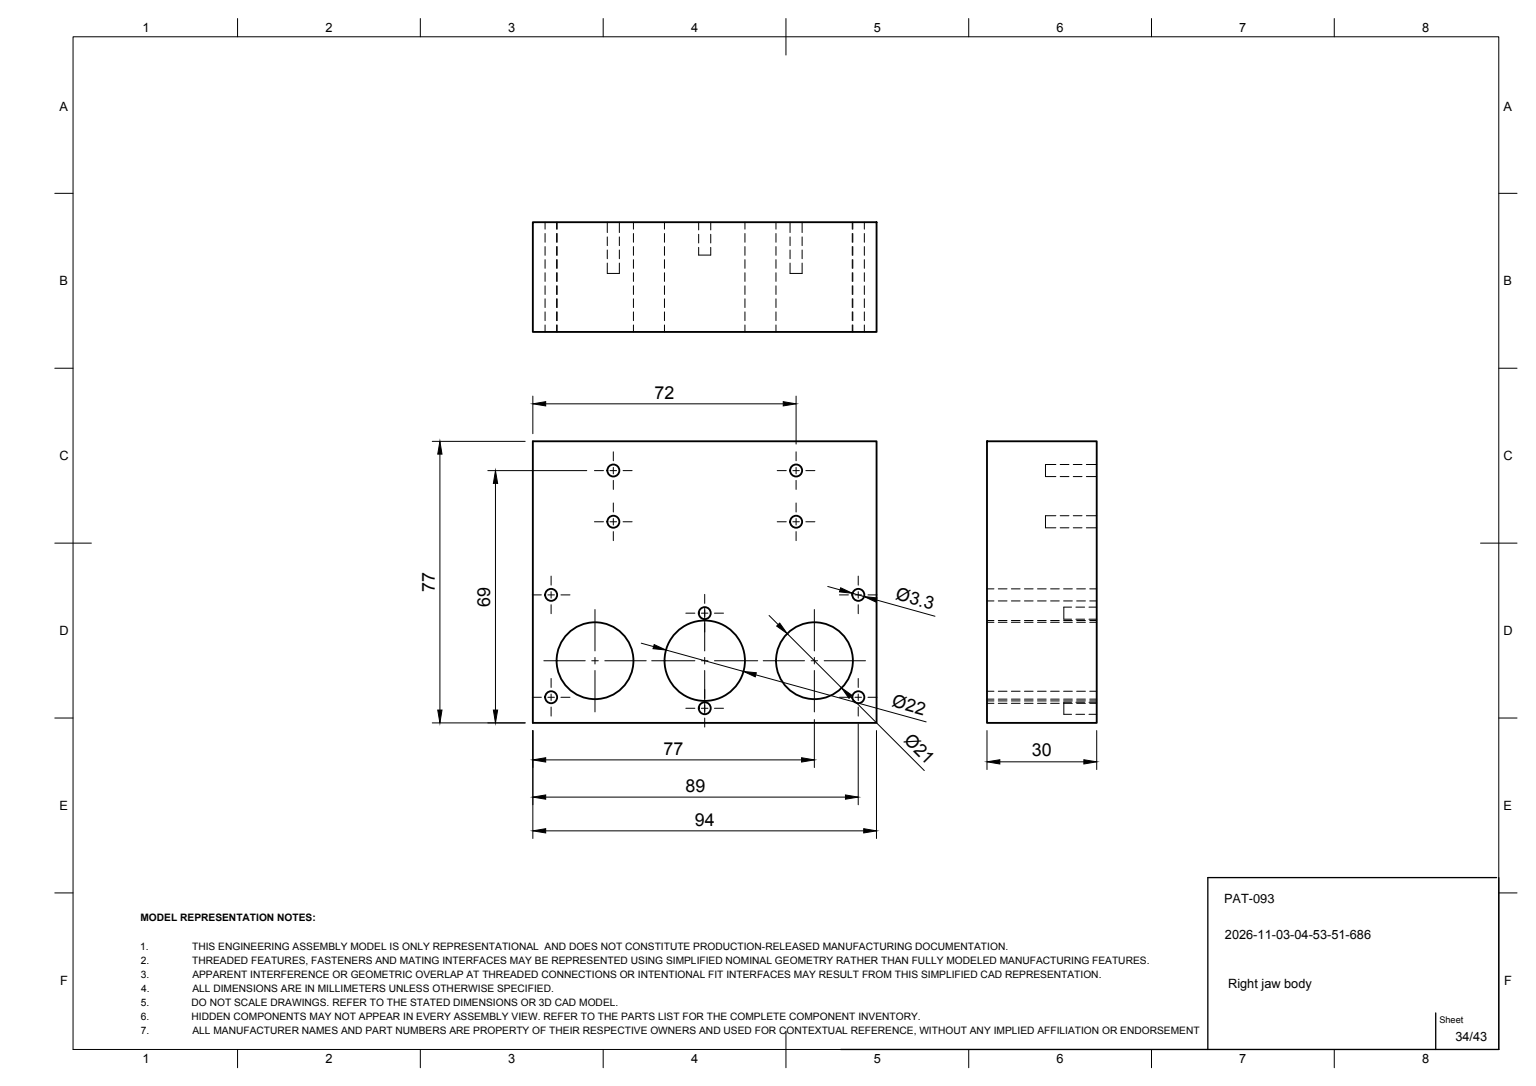
ISO-10303-21;
HEADER;
/* Generated by software containing ST-Developer
 * from STEP Tools, Inc. (www.steptools.com) 
 */

FILE_DESCRIPTION(
/* description */ ('Self-centering screw clamp'),
/* implementation_level */ '2;1');

FILE_NAME(
/* name */ 'Right jaw body.step',
/* time_stamp */ '2026-10-28T03:25:31-07:00',
/* author */ (''),
/* organization */ (''),
/* preprocessor_version */ 'ST-DEVELOPER v20.2',
/* originating_system */ 'Autodesk Translation Framework v15.17.0.0',
/* authorisation */ '');

FILE_SCHEMA (('AUTOMOTIVE_DESIGN { 1 0 10303 214 3 1 1 }'));
ENDSEC;

DATA;
#10=MECHANICAL_DESIGN_GEOMETRIC_PRESENTATION_REPRESENTATION('',(#655),#16799);
#566=SHAPE_REPRESENTATION_RELATIONSHIP('SRR','None',#17042,#607);
#607=ADVANCED_BREP_SHAPE_REPRESENTATION('',(#703),#16780);
#655=STYLED_ITEM('',(#17305),#703);
#703=MANIFOLD_SOLID_BREP('Body1',#9106);
#916=FACE_BOUND('',#2304,.T.);
#917=FACE_BOUND('',#2305,.T.);
#918=FACE_BOUND('',#2306,.T.);
#919=FACE_BOUND('',#2307,.T.);
#920=FACE_BOUND('',#2308,.T.);
#921=FACE_BOUND('',#2309,.T.);
#922=FACE_BOUND('',#2310,.T.);
#923=FACE_BOUND('',#2313,.T.);
#924=FACE_BOUND('',#2314,.T.);
#925=FACE_BOUND('',#2315,.T.);
#926=FACE_BOUND('',#2316,.T.);
#927=FACE_BOUND('',#2317,.T.);
#928=FACE_BOUND('',#2318,.T.);
#929=FACE_BOUND('',#2319,.T.);
#930=FACE_BOUND('',#2320,.T.);
#931=FACE_BOUND('',#2321,.T.);
#932=FACE_BOUND('',#2322,.T.);
#933=FACE_BOUND('',#2323,.T.);
#934=FACE_BOUND('',#2324,.T.);
#935=FACE_BOUND('',#2325,.T.);
#1161=PLANE('',#10260);
#1162=PLANE('',#10264);
#1163=PLANE('',#10268);
#1164=PLANE('',#10272);
#1165=PLANE('',#10276);
#1166=PLANE('',#10280);
#1167=PLANE('',#10302);
#1168=PLANE('',#10303);
#1169=PLANE('',#10304);
#1170=PLANE('',#10305);
#1171=PLANE('',#10306);
#1172=PLANE('',#10307);
#1581=FACE_OUTER_BOUND('',#2283,.T.);
#1582=FACE_OUTER_BOUND('',#2284,.T.);
#1583=FACE_OUTER_BOUND('',#2285,.T.);
#1584=FACE_OUTER_BOUND('',#2286,.T.);
#1585=FACE_OUTER_BOUND('',#2287,.T.);
#1586=FACE_OUTER_BOUND('',#2288,.T.);
#1587=FACE_OUTER_BOUND('',#2289,.T.);
#1588=FACE_OUTER_BOUND('',#2290,.T.);
#1589=FACE_OUTER_BOUND('',#2291,.T.);
#1590=FACE_OUTER_BOUND('',#2292,.T.);
#1591=FACE_OUTER_BOUND('',#2293,.T.);
#1592=FACE_OUTER_BOUND('',#2294,.T.);
#1593=FACE_OUTER_BOUND('',#2295,.T.);
#1594=FACE_OUTER_BOUND('',#2296,.T.);
#1595=FACE_OUTER_BOUND('',#2297,.T.);
#1596=FACE_OUTER_BOUND('',#2298,.T.);
#1597=FACE_OUTER_BOUND('',#2299,.T.);
#1598=FACE_OUTER_BOUND('',#2300,.T.);
#1599=FACE_OUTER_BOUND('',#2301,.T.);
#1600=FACE_OUTER_BOUND('',#2302,.T.);
#1601=FACE_OUTER_BOUND('',#2303,.T.);
#1602=FACE_OUTER_BOUND('',#2311,.T.);
#1603=FACE_OUTER_BOUND('',#2312,.T.);
#1604=FACE_OUTER_BOUND('',#2326,.T.);
#1605=FACE_OUTER_BOUND('',#2327,.T.);
#2283=EDGE_LOOP('',(#7551,#7552,#7553,#7554));
#2284=EDGE_LOOP('',(#7555));
#2285=EDGE_LOOP('',(#7556,#7557,#7558,#7559));
#2286=EDGE_LOOP('',(#7560));
#2287=EDGE_LOOP('',(#7561,#7562,#7563,#7564));
#2288=EDGE_LOOP('',(#7565));
#2289=EDGE_LOOP('',(#7566,#7567,#7568,#7569));
#2290=EDGE_LOOP('',(#7570));
#2291=EDGE_LOOP('',(#7571,#7572,#7573,#7574));
#2292=EDGE_LOOP('',(#7575));
#2293=EDGE_LOOP('',(#7576,#7577,#7578,#7579));
#2294=EDGE_LOOP('',(#7580));
#2295=EDGE_LOOP('',(#7581,#7582,#7583,#7584));
#2296=EDGE_LOOP('',(#7585,#7586,#7587,#7588));
#2297=EDGE_LOOP('',(#7589,#7590,#7591,#7592));
#2298=EDGE_LOOP('',(#7593,#7594,#7595,#7596));
#2299=EDGE_LOOP('',(#7597,#7598,#7599,#7600));
#2300=EDGE_LOOP('',(#7601,#7602,#7603,#7604));
#2301=EDGE_LOOP('',(#7605,#7606,#7607,#7608));
#2302=EDGE_LOOP('',(#7609,#7610,#7611,#7612));
#2303=EDGE_LOOP('',(#7613,#7614,#7615,#7616));
#2304=EDGE_LOOP('',(#7617));
#2305=EDGE_LOOP('',(#7618));
#2306=EDGE_LOOP('',(#7619));
#2307=EDGE_LOOP('',(#7620));
#2308=EDGE_LOOP('',(#7621));
#2309=EDGE_LOOP('',(#7622));
#2310=EDGE_LOOP('',(#7623));
#2311=EDGE_LOOP('',(#7624,#7625,#7626,#7627));
#2312=EDGE_LOOP('',(#7628,#7629,#7630,#7631));
#2313=EDGE_LOOP('',(#7632));
#2314=EDGE_LOOP('',(#7633));
#2315=EDGE_LOOP('',(#7634));
#2316=EDGE_LOOP('',(#7635));
#2317=EDGE_LOOP('',(#7636));
#2318=EDGE_LOOP('',(#7637));
#2319=EDGE_LOOP('',(#7638));
#2320=EDGE_LOOP('',(#7639));
#2321=EDGE_LOOP('',(#7640));
#2322=EDGE_LOOP('',(#7641));
#2323=EDGE_LOOP('',(#7642));
#2324=EDGE_LOOP('',(#7643));
#2325=EDGE_LOOP('',(#7644));
#2326=EDGE_LOOP('',(#7645,#7646,#7647,#7648));
#2327=EDGE_LOOP('',(#7649,#7650,#7651,#7652));
#2934=LINE('',#15598,#3507);
#2935=LINE('',#15605,#3508);
#2936=LINE('',#15612,#3509);
#2937=LINE('',#15619,#3510);
#2938=LINE('',#15626,#3511);
#2939=LINE('',#15633,#3512);
#2940=LINE('',#15640,#3513);
#2941=LINE('',#15646,#3514);
#2942=LINE('',#15652,#3515);
#2943=LINE('',#15658,#3516);
#2944=LINE('',#15664,#3517);
#2945=LINE('',#15670,#3518);
#2946=LINE('',#15676,#3519);
#2947=LINE('',#15681,#3520);
#2948=LINE('',#15683,#3521);
#2949=LINE('',#15685,#3522);
#2950=LINE('',#15686,#3523);
#2951=LINE('',#15689,#3524);
#2952=LINE('',#15691,#3525);
#2953=LINE('',#15692,#3526);
#2954=LINE('',#15695,#3527);
#2955=LINE('',#15697,#3528);
#2956=LINE('',#15698,#3529);
#2957=LINE('',#15700,#3530);
#2958=LINE('',#15701,#3531);
#3507=VECTOR('',#12473,0.165);
#3508=VECTOR('',#12482,0.164999999999999);
#3509=VECTOR('',#12491,0.165);
#3510=VECTOR('',#12500,0.164999999999999);
#3511=VECTOR('',#12509,0.165);
#3512=VECTOR('',#12518,0.165);
#3513=VECTOR('',#12527,0.165);
#3514=VECTOR('',#12534,0.165);
#3515=VECTOR('',#12541,0.165);
#3516=VECTOR('',#12548,0.165);
#3517=VECTOR('',#12555,1.1);
#3518=VECTOR('',#12562,1.05);
#3519=VECTOR('',#12569,1.05);
#3520=VECTOR('',#12574,1.);
#3521=VECTOR('',#12575,1.);
#3522=VECTOR('',#12576,1.);
#3523=VECTOR('',#12577,1.);
#3524=VECTOR('',#12580,1.);
#3525=VECTOR('',#12581,1.);
#3526=VECTOR('',#12582,1.);
#3527=VECTOR('',#12585,1.);
#3528=VECTOR('',#12586,1.);
#3529=VECTOR('',#12587,1.);
#3530=VECTOR('',#12590,1.);
#3531=VECTOR('',#12591,1.);
#4060=CIRCLE('',#10258,0.165);
#4061=CIRCLE('',#10259,0.165);
#4062=CIRCLE('',#10262,0.164999999999999);
#4063=CIRCLE('',#10263,0.164999999999999);
#4064=CIRCLE('',#10266,0.165);
#4065=CIRCLE('',#10267,0.165);
#4066=CIRCLE('',#10270,0.164999999999999);
#4067=CIRCLE('',#10271,0.164999999999999);
#4068=CIRCLE('',#10274,0.165);
#4069=CIRCLE('',#10275,0.165);
#4070=CIRCLE('',#10278,0.165);
#4071=CIRCLE('',#10279,0.165);
#4072=CIRCLE('',#10282,0.165);
#4073=CIRCLE('',#10283,0.165);
#4074=CIRCLE('',#10285,0.165);
#4075=CIRCLE('',#10286,0.165);
#4076=CIRCLE('',#10288,0.165);
#4077=CIRCLE('',#10289,0.165);
#4078=CIRCLE('',#10291,0.165);
#4079=CIRCLE('',#10292,0.165);
#4080=CIRCLE('',#10294,1.1);
#4081=CIRCLE('',#10295,1.1);
#4082=CIRCLE('',#10297,1.05);
#4083=CIRCLE('',#10298,1.05);
#4084=CIRCLE('',#10300,1.05);
#4085=CIRCLE('',#10301,1.05);
#4711=VERTEX_POINT('',#15595);
#4712=VERTEX_POINT('',#15597);
#4713=VERTEX_POINT('',#15602);
#4714=VERTEX_POINT('',#15604);
#4715=VERTEX_POINT('',#15609);
#4716=VERTEX_POINT('',#15611);
#4717=VERTEX_POINT('',#15616);
#4718=VERTEX_POINT('',#15618);
#4719=VERTEX_POINT('',#15623);
#4720=VERTEX_POINT('',#15625);
#4721=VERTEX_POINT('',#15630);
#4722=VERTEX_POINT('',#15632);
#4723=VERTEX_POINT('',#15637);
#4724=VERTEX_POINT('',#15639);
#4725=VERTEX_POINT('',#15643);
#4726=VERTEX_POINT('',#15645);
#4727=VERTEX_POINT('',#15649);
#4728=VERTEX_POINT('',#15651);
#4729=VERTEX_POINT('',#15655);
#4730=VERTEX_POINT('',#15657);
#4731=VERTEX_POINT('',#15661);
#4732=VERTEX_POINT('',#15663);
#4733=VERTEX_POINT('',#15667);
#4734=VERTEX_POINT('',#15669);
#4735=VERTEX_POINT('',#15673);
#4736=VERTEX_POINT('',#15675);
#4737=VERTEX_POINT('',#15679);
#4738=VERTEX_POINT('',#15680);
#4739=VERTEX_POINT('',#15682);
#4740=VERTEX_POINT('',#15684);
#4741=VERTEX_POINT('',#15688);
#4742=VERTEX_POINT('',#15690);
#4743=VERTEX_POINT('',#15694);
#4744=VERTEX_POINT('',#15696);
#5700=EDGE_CURVE('',#4711,#4711,#4060,.T.);
#5701=EDGE_CURVE('',#4711,#4712,#2934,.T.);
#5702=EDGE_CURVE('',#4712,#4712,#4061,.T.);
#5703=EDGE_CURVE('',#4713,#4713,#4062,.T.);
#5704=EDGE_CURVE('',#4713,#4714,#2935,.T.);
#5705=EDGE_CURVE('',#4714,#4714,#4063,.T.);
#5706=EDGE_CURVE('',#4715,#4715,#4064,.T.);
#5707=EDGE_CURVE('',#4715,#4716,#2936,.T.);
#5708=EDGE_CURVE('',#4716,#4716,#4065,.T.);
#5709=EDGE_CURVE('',#4717,#4717,#4066,.T.);
#5710=EDGE_CURVE('',#4717,#4718,#2937,.T.);
#5711=EDGE_CURVE('',#4718,#4718,#4067,.T.);
#5712=EDGE_CURVE('',#4719,#4719,#4068,.T.);
#5713=EDGE_CURVE('',#4719,#4720,#2938,.T.);
#5714=EDGE_CURVE('',#4720,#4720,#4069,.T.);
#5715=EDGE_CURVE('',#4721,#4721,#4070,.T.);
#5716=EDGE_CURVE('',#4721,#4722,#2939,.T.);
#5717=EDGE_CURVE('',#4722,#4722,#4071,.T.);
#5718=EDGE_CURVE('',#4723,#4723,#4072,.T.);
#5719=EDGE_CURVE('',#4723,#4724,#2940,.T.);
#5720=EDGE_CURVE('',#4724,#4724,#4073,.T.);
#5721=EDGE_CURVE('',#4725,#4725,#4074,.T.);
#5722=EDGE_CURVE('',#4725,#4726,#2941,.T.);
#5723=EDGE_CURVE('',#4726,#4726,#4075,.T.);
#5724=EDGE_CURVE('',#4727,#4727,#4076,.T.);
#5725=EDGE_CURVE('',#4727,#4728,#2942,.T.);
#5726=EDGE_CURVE('',#4728,#4728,#4077,.T.);
#5727=EDGE_CURVE('',#4729,#4729,#4078,.T.);
#5728=EDGE_CURVE('',#4729,#4730,#2943,.T.);
#5729=EDGE_CURVE('',#4730,#4730,#4079,.T.);
#5730=EDGE_CURVE('',#4731,#4731,#4080,.T.);
#5731=EDGE_CURVE('',#4731,#4732,#2944,.T.);
#5732=EDGE_CURVE('',#4732,#4732,#4081,.T.);
#5733=EDGE_CURVE('',#4733,#4733,#4082,.T.);
#5734=EDGE_CURVE('',#4733,#4734,#2945,.T.);
#5735=EDGE_CURVE('',#4734,#4734,#4083,.T.);
#5736=EDGE_CURVE('',#4735,#4735,#4084,.T.);
#5737=EDGE_CURVE('',#4735,#4736,#2946,.T.);
#5738=EDGE_CURVE('',#4736,#4736,#4085,.T.);
#5739=EDGE_CURVE('',#4737,#4738,#2947,.T.);
#5740=EDGE_CURVE('',#4738,#4739,#2948,.T.);
#5741=EDGE_CURVE('',#4740,#4739,#2949,.T.);
#5742=EDGE_CURVE('',#4737,#4740,#2950,.T.);
#5743=EDGE_CURVE('',#4741,#4737,#2951,.T.);
#5744=EDGE_CURVE('',#4742,#4740,#2952,.T.);
#5745=EDGE_CURVE('',#4741,#4742,#2953,.T.);
#5746=EDGE_CURVE('',#4743,#4741,#2954,.T.);
#5747=EDGE_CURVE('',#4744,#4742,#2955,.T.);
#5748=EDGE_CURVE('',#4743,#4744,#2956,.T.);
#5749=EDGE_CURVE('',#4738,#4743,#2957,.T.);
#5750=EDGE_CURVE('',#4739,#4744,#2958,.T.);
#7551=ORIENTED_EDGE('',*,*,#5700,.F.);
#7552=ORIENTED_EDGE('',*,*,#5701,.T.);
#7553=ORIENTED_EDGE('',*,*,#5702,.T.);
#7554=ORIENTED_EDGE('',*,*,#5701,.F.);
#7555=ORIENTED_EDGE('',*,*,#5702,.F.);
#7556=ORIENTED_EDGE('',*,*,#5703,.F.);
#7557=ORIENTED_EDGE('',*,*,#5704,.T.);
#7558=ORIENTED_EDGE('',*,*,#5705,.T.);
#7559=ORIENTED_EDGE('',*,*,#5704,.F.);
#7560=ORIENTED_EDGE('',*,*,#5705,.F.);
#7561=ORIENTED_EDGE('',*,*,#5706,.F.);
#7562=ORIENTED_EDGE('',*,*,#5707,.T.);
#7563=ORIENTED_EDGE('',*,*,#5708,.T.);
#7564=ORIENTED_EDGE('',*,*,#5707,.F.);
#7565=ORIENTED_EDGE('',*,*,#5708,.F.);
#7566=ORIENTED_EDGE('',*,*,#5709,.F.);
#7567=ORIENTED_EDGE('',*,*,#5710,.T.);
#7568=ORIENTED_EDGE('',*,*,#5711,.T.);
#7569=ORIENTED_EDGE('',*,*,#5710,.F.);
#7570=ORIENTED_EDGE('',*,*,#5711,.F.);
#7571=ORIENTED_EDGE('',*,*,#5712,.F.);
#7572=ORIENTED_EDGE('',*,*,#5713,.T.);
#7573=ORIENTED_EDGE('',*,*,#5714,.T.);
#7574=ORIENTED_EDGE('',*,*,#5713,.F.);
#7575=ORIENTED_EDGE('',*,*,#5714,.F.);
#7576=ORIENTED_EDGE('',*,*,#5715,.F.);
#7577=ORIENTED_EDGE('',*,*,#5716,.T.);
#7578=ORIENTED_EDGE('',*,*,#5717,.T.);
#7579=ORIENTED_EDGE('',*,*,#5716,.F.);
#7580=ORIENTED_EDGE('',*,*,#5717,.F.);
#7581=ORIENTED_EDGE('',*,*,#5718,.F.);
#7582=ORIENTED_EDGE('',*,*,#5719,.T.);
#7583=ORIENTED_EDGE('',*,*,#5720,.F.);
#7584=ORIENTED_EDGE('',*,*,#5719,.F.);
#7585=ORIENTED_EDGE('',*,*,#5721,.F.);
#7586=ORIENTED_EDGE('',*,*,#5722,.T.);
#7587=ORIENTED_EDGE('',*,*,#5723,.F.);
#7588=ORIENTED_EDGE('',*,*,#5722,.F.);
#7589=ORIENTED_EDGE('',*,*,#5724,.F.);
#7590=ORIENTED_EDGE('',*,*,#5725,.T.);
#7591=ORIENTED_EDGE('',*,*,#5726,.F.);
#7592=ORIENTED_EDGE('',*,*,#5725,.F.);
#7593=ORIENTED_EDGE('',*,*,#5727,.F.);
#7594=ORIENTED_EDGE('',*,*,#5728,.T.);
#7595=ORIENTED_EDGE('',*,*,#5729,.F.);
#7596=ORIENTED_EDGE('',*,*,#5728,.F.);
#7597=ORIENTED_EDGE('',*,*,#5730,.F.);
#7598=ORIENTED_EDGE('',*,*,#5731,.T.);
#7599=ORIENTED_EDGE('',*,*,#5732,.F.);
#7600=ORIENTED_EDGE('',*,*,#5731,.F.);
#7601=ORIENTED_EDGE('',*,*,#5733,.F.);
#7602=ORIENTED_EDGE('',*,*,#5734,.T.);
#7603=ORIENTED_EDGE('',*,*,#5735,.F.);
#7604=ORIENTED_EDGE('',*,*,#5734,.F.);
#7605=ORIENTED_EDGE('',*,*,#5736,.F.);
#7606=ORIENTED_EDGE('',*,*,#5737,.T.);
#7607=ORIENTED_EDGE('',*,*,#5738,.F.);
#7608=ORIENTED_EDGE('',*,*,#5737,.F.);
#7609=ORIENTED_EDGE('',*,*,#5739,.T.);
#7610=ORIENTED_EDGE('',*,*,#5740,.T.);
#7611=ORIENTED_EDGE('',*,*,#5741,.F.);
#7612=ORIENTED_EDGE('',*,*,#5742,.F.);
#7613=ORIENTED_EDGE('',*,*,#5743,.T.);
#7614=ORIENTED_EDGE('',*,*,#5742,.T.);
#7615=ORIENTED_EDGE('',*,*,#5744,.F.);
#7616=ORIENTED_EDGE('',*,*,#5745,.F.);
#7617=ORIENTED_EDGE('',*,*,#5738,.T.);
#7618=ORIENTED_EDGE('',*,*,#5735,.T.);
#7619=ORIENTED_EDGE('',*,*,#5732,.T.);
#7620=ORIENTED_EDGE('',*,*,#5729,.T.);
#7621=ORIENTED_EDGE('',*,*,#5726,.T.);
#7622=ORIENTED_EDGE('',*,*,#5723,.T.);
#7623=ORIENTED_EDGE('',*,*,#5720,.T.);
#7624=ORIENTED_EDGE('',*,*,#5746,.T.);
#7625=ORIENTED_EDGE('',*,*,#5745,.T.);
#7626=ORIENTED_EDGE('',*,*,#5747,.F.);
#7627=ORIENTED_EDGE('',*,*,#5748,.F.);
#7628=ORIENTED_EDGE('',*,*,#5749,.T.);
#7629=ORIENTED_EDGE('',*,*,#5748,.T.);
#7630=ORIENTED_EDGE('',*,*,#5750,.F.);
#7631=ORIENTED_EDGE('',*,*,#5740,.F.);
#7632=ORIENTED_EDGE('',*,*,#5712,.T.);
#7633=ORIENTED_EDGE('',*,*,#5715,.T.);
#7634=ORIENTED_EDGE('',*,*,#5736,.T.);
#7635=ORIENTED_EDGE('',*,*,#5733,.T.);
#7636=ORIENTED_EDGE('',*,*,#5730,.T.);
#7637=ORIENTED_EDGE('',*,*,#5727,.T.);
#7638=ORIENTED_EDGE('',*,*,#5724,.T.);
#7639=ORIENTED_EDGE('',*,*,#5721,.T.);
#7640=ORIENTED_EDGE('',*,*,#5718,.T.);
#7641=ORIENTED_EDGE('',*,*,#5709,.T.);
#7642=ORIENTED_EDGE('',*,*,#5706,.T.);
#7643=ORIENTED_EDGE('',*,*,#5703,.T.);
#7644=ORIENTED_EDGE('',*,*,#5700,.T.);
#7645=ORIENTED_EDGE('',*,*,#5750,.T.);
#7646=ORIENTED_EDGE('',*,*,#5747,.T.);
#7647=ORIENTED_EDGE('',*,*,#5744,.T.);
#7648=ORIENTED_EDGE('',*,*,#5741,.T.);
#7649=ORIENTED_EDGE('',*,*,#5749,.F.);
#7650=ORIENTED_EDGE('',*,*,#5739,.F.);
#7651=ORIENTED_EDGE('',*,*,#5743,.F.);
#7652=ORIENTED_EDGE('',*,*,#5746,.F.);
#8496=CYLINDRICAL_SURFACE('',#10257,0.165);
#8497=CYLINDRICAL_SURFACE('',#10261,0.164999999999999);
#8498=CYLINDRICAL_SURFACE('',#10265,0.165);
#8499=CYLINDRICAL_SURFACE('',#10269,0.164999999999999);
#8500=CYLINDRICAL_SURFACE('',#10273,0.165);
#8501=CYLINDRICAL_SURFACE('',#10277,0.165);
#8502=CYLINDRICAL_SURFACE('',#10281,0.165);
#8503=CYLINDRICAL_SURFACE('',#10284,0.165);
#8504=CYLINDRICAL_SURFACE('',#10287,0.165);
#8505=CYLINDRICAL_SURFACE('',#10290,0.165);
#8506=CYLINDRICAL_SURFACE('',#10293,1.1);
#8507=CYLINDRICAL_SURFACE('',#10296,1.05);
#8508=CYLINDRICAL_SURFACE('',#10299,1.05);
#8879=ADVANCED_FACE('',(#1581),#8496,.F.);
#8880=ADVANCED_FACE('',(#1582),#1161,.F.);
#8881=ADVANCED_FACE('',(#1583),#8497,.F.);
#8882=ADVANCED_FACE('',(#1584),#1162,.F.);
#8883=ADVANCED_FACE('',(#1585),#8498,.F.);
#8884=ADVANCED_FACE('',(#1586),#1163,.F.);
#8885=ADVANCED_FACE('',(#1587),#8499,.F.);
#8886=ADVANCED_FACE('',(#1588),#1164,.F.);
#8887=ADVANCED_FACE('',(#1589),#8500,.F.);
#8888=ADVANCED_FACE('',(#1590),#1165,.F.);
#8889=ADVANCED_FACE('',(#1591),#8501,.F.);
#8890=ADVANCED_FACE('',(#1592),#1166,.F.);
#8891=ADVANCED_FACE('',(#1593),#8502,.F.);
#8892=ADVANCED_FACE('',(#1594),#8503,.F.);
#8893=ADVANCED_FACE('',(#1595),#8504,.F.);
#8894=ADVANCED_FACE('',(#1596),#8505,.F.);
#8895=ADVANCED_FACE('',(#1597),#8506,.F.);
#8896=ADVANCED_FACE('',(#1598),#8507,.F.);
#8897=ADVANCED_FACE('',(#1599),#8508,.F.);
#8898=ADVANCED_FACE('',(#1600),#1167,.T.);
#8899=ADVANCED_FACE('',(#1601,#916,#917,#918,#919,#920,#921,#922),#1168,
 .T.);
#8900=ADVANCED_FACE('',(#1602),#1169,.T.);
#8901=ADVANCED_FACE('',(#1603,#923,#924,#925,#926,#927,#928,#929,#930,#931,
#932,#933,#934,#935),#1170,.T.);
#8902=ADVANCED_FACE('',(#1604),#1171,.T.);
#8903=ADVANCED_FACE('',(#1605),#1172,.F.);
#9106=CLOSED_SHELL('',(#8879,#8880,#8881,#8882,#8883,#8884,#8885,#8886,
#8887,#8888,#8889,#8890,#8891,#8892,#8893,#8894,#8895,#8896,#8897,#8898,
#8899,#8900,#8901,#8902,#8903));
#10256=AXIS2_PLACEMENT_3D('',#15593,#12467,#12468);
#10257=AXIS2_PLACEMENT_3D('',#15594,#12469,#12470);
#10258=AXIS2_PLACEMENT_3D('',#15596,#12471,#12472);
#10259=AXIS2_PLACEMENT_3D('',#15599,#12474,#12475);
#10260=AXIS2_PLACEMENT_3D('',#15600,#12476,#12477);
#10261=AXIS2_PLACEMENT_3D('',#15601,#12478,#12479);
#10262=AXIS2_PLACEMENT_3D('',#15603,#12480,#12481);
#10263=AXIS2_PLACEMENT_3D('',#15606,#12483,#12484);
#10264=AXIS2_PLACEMENT_3D('',#15607,#12485,#12486);
#10265=AXIS2_PLACEMENT_3D('',#15608,#12487,#12488);
#10266=AXIS2_PLACEMENT_3D('',#15610,#12489,#12490);
#10267=AXIS2_PLACEMENT_3D('',#15613,#12492,#12493);
#10268=AXIS2_PLACEMENT_3D('',#15614,#12494,#12495);
#10269=AXIS2_PLACEMENT_3D('',#15615,#12496,#12497);
#10270=AXIS2_PLACEMENT_3D('',#15617,#12498,#12499);
#10271=AXIS2_PLACEMENT_3D('',#15620,#12501,#12502);
#10272=AXIS2_PLACEMENT_3D('',#15621,#12503,#12504);
#10273=AXIS2_PLACEMENT_3D('',#15622,#12505,#12506);
#10274=AXIS2_PLACEMENT_3D('',#15624,#12507,#12508);
#10275=AXIS2_PLACEMENT_3D('',#15627,#12510,#12511);
#10276=AXIS2_PLACEMENT_3D('',#15628,#12512,#12513);
#10277=AXIS2_PLACEMENT_3D('',#15629,#12514,#12515);
#10278=AXIS2_PLACEMENT_3D('',#15631,#12516,#12517);
#10279=AXIS2_PLACEMENT_3D('',#15634,#12519,#12520);
#10280=AXIS2_PLACEMENT_3D('',#15635,#12521,#12522);
#10281=AXIS2_PLACEMENT_3D('',#15636,#12523,#12524);
#10282=AXIS2_PLACEMENT_3D('',#15638,#12525,#12526);
#10283=AXIS2_PLACEMENT_3D('',#15641,#12528,#12529);
#10284=AXIS2_PLACEMENT_3D('',#15642,#12530,#12531);
#10285=AXIS2_PLACEMENT_3D('',#15644,#12532,#12533);
#10286=AXIS2_PLACEMENT_3D('',#15647,#12535,#12536);
#10287=AXIS2_PLACEMENT_3D('',#15648,#12537,#12538);
#10288=AXIS2_PLACEMENT_3D('',#15650,#12539,#12540);
#10289=AXIS2_PLACEMENT_3D('',#15653,#12542,#12543);
#10290=AXIS2_PLACEMENT_3D('',#15654,#12544,#12545);
#10291=AXIS2_PLACEMENT_3D('',#15656,#12546,#12547);
#10292=AXIS2_PLACEMENT_3D('',#15659,#12549,#12550);
#10293=AXIS2_PLACEMENT_3D('',#15660,#12551,#12552);
#10294=AXIS2_PLACEMENT_3D('',#15662,#12553,#12554);
#10295=AXIS2_PLACEMENT_3D('',#15665,#12556,#12557);
#10296=AXIS2_PLACEMENT_3D('',#15666,#12558,#12559);
#10297=AXIS2_PLACEMENT_3D('',#15668,#12560,#12561);
#10298=AXIS2_PLACEMENT_3D('',#15671,#12563,#12564);
#10299=AXIS2_PLACEMENT_3D('',#15672,#12565,#12566);
#10300=AXIS2_PLACEMENT_3D('',#15674,#12567,#12568);
#10301=AXIS2_PLACEMENT_3D('',#15677,#12570,#12571);
#10302=AXIS2_PLACEMENT_3D('',#15678,#12572,#12573);
#10303=AXIS2_PLACEMENT_3D('',#15687,#12578,#12579);
#10304=AXIS2_PLACEMENT_3D('',#15693,#12583,#12584);
#10305=AXIS2_PLACEMENT_3D('',#15699,#12588,#12589);
#10306=AXIS2_PLACEMENT_3D('',#15702,#12592,#12593);
#10307=AXIS2_PLACEMENT_3D('',#15703,#12594,#12595);
#12467=DIRECTION('axis',(0.,0.,1.));
#12468=DIRECTION('refdir',(1.,0.,0.));
#12469=DIRECTION('center_axis',(1.,0.,0.));
#12470=DIRECTION('ref_axis',(0.,0.,-1.));
#12471=DIRECTION('center_axis',(1.,0.,0.));
#12472=DIRECTION('ref_axis',(0.,0.,-1.));
#12473=DIRECTION('',(1.,0.,0.));
#12474=DIRECTION('center_axis',(1.,0.,0.));
#12475=DIRECTION('ref_axis',(0.,0.,-1.));
#12476=DIRECTION('center_axis',(1.,0.,0.));
#12477=DIRECTION('ref_axis',(0.,0.,-1.));
#12478=DIRECTION('center_axis',(1.,0.,0.));
#12479=DIRECTION('ref_axis',(0.,0.,-1.));
#12480=DIRECTION('center_axis',(1.,0.,0.));
#12481=DIRECTION('ref_axis',(0.,0.,-1.));
#12482=DIRECTION('',(1.,0.,0.));
#12483=DIRECTION('center_axis',(1.,0.,0.));
#12484=DIRECTION('ref_axis',(0.,0.,-1.));
#12485=DIRECTION('center_axis',(1.,0.,0.));
#12486=DIRECTION('ref_axis',(0.,0.,-1.));
#12487=DIRECTION('center_axis',(1.,0.,0.));
#12488=DIRECTION('ref_axis',(0.,0.,-1.));
#12489=DIRECTION('center_axis',(1.,0.,0.));
#12490=DIRECTION('ref_axis',(0.,0.,-1.));
#12491=DIRECTION('',(1.,0.,0.));
#12492=DIRECTION('center_axis',(1.,0.,0.));
#12493=DIRECTION('ref_axis',(0.,0.,-1.));
#12494=DIRECTION('center_axis',(1.,0.,0.));
#12495=DIRECTION('ref_axis',(0.,0.,-1.));
#12496=DIRECTION('center_axis',(1.,0.,0.));
#12497=DIRECTION('ref_axis',(0.,0.,-1.));
#12498=DIRECTION('center_axis',(1.,0.,0.));
#12499=DIRECTION('ref_axis',(0.,0.,-1.));
#12500=DIRECTION('',(1.,0.,0.));
#12501=DIRECTION('center_axis',(1.,0.,0.));
#12502=DIRECTION('ref_axis',(0.,0.,-1.));
#12503=DIRECTION('center_axis',(1.,0.,0.));
#12504=DIRECTION('ref_axis',(0.,0.,-1.));
#12505=DIRECTION('center_axis',(1.,0.,0.));
#12506=DIRECTION('ref_axis',(0.,0.,-1.));
#12507=DIRECTION('center_axis',(1.,0.,0.));
#12508=DIRECTION('ref_axis',(0.,0.,-1.));
#12509=DIRECTION('',(1.,0.,0.));
#12510=DIRECTION('center_axis',(1.,0.,0.));
#12511=DIRECTION('ref_axis',(0.,0.,-1.));
#12512=DIRECTION('center_axis',(1.,0.,0.));
#12513=DIRECTION('ref_axis',(0.,0.,-1.));
#12514=DIRECTION('center_axis',(1.,0.,0.));
#12515=DIRECTION('ref_axis',(0.,0.,-1.));
#12516=DIRECTION('center_axis',(1.,0.,0.));
#12517=DIRECTION('ref_axis',(0.,0.,-1.));
#12518=DIRECTION('',(1.,0.,0.));
#12519=DIRECTION('center_axis',(1.,0.,0.));
#12520=DIRECTION('ref_axis',(0.,0.,-1.));
#12521=DIRECTION('center_axis',(1.,0.,0.));
#12522=DIRECTION('ref_axis',(0.,0.,-1.));
#12523=DIRECTION('center_axis',(1.,0.,0.));
#12524=DIRECTION('ref_axis',(0.,0.,-1.));
#12525=DIRECTION('center_axis',(1.,0.,0.));
#12526=DIRECTION('ref_axis',(0.,0.,-1.));
#12527=DIRECTION('',(1.,0.,0.));
#12528=DIRECTION('center_axis',(-1.,0.,0.));
#12529=DIRECTION('ref_axis',(0.,0.,-1.));
#12530=DIRECTION('center_axis',(1.,0.,0.));
#12531=DIRECTION('ref_axis',(0.,0.,-1.));
#12532=DIRECTION('center_axis',(1.,0.,0.));
#12533=DIRECTION('ref_axis',(0.,0.,-1.));
#12534=DIRECTION('',(1.,0.,0.));
#12535=DIRECTION('center_axis',(-1.,0.,0.));
#12536=DIRECTION('ref_axis',(0.,0.,-1.));
#12537=DIRECTION('center_axis',(1.,0.,0.));
#12538=DIRECTION('ref_axis',(0.,0.,-1.));
#12539=DIRECTION('center_axis',(1.,0.,0.));
#12540=DIRECTION('ref_axis',(0.,0.,-1.));
#12541=DIRECTION('',(1.,0.,0.));
#12542=DIRECTION('center_axis',(-1.,0.,0.));
#12543=DIRECTION('ref_axis',(0.,0.,-1.));
#12544=DIRECTION('center_axis',(1.,0.,0.));
#12545=DIRECTION('ref_axis',(0.,0.,-1.));
#12546=DIRECTION('center_axis',(1.,0.,0.));
#12547=DIRECTION('ref_axis',(0.,0.,-1.));
#12548=DIRECTION('',(1.,0.,0.));
#12549=DIRECTION('center_axis',(-1.,0.,0.));
#12550=DIRECTION('ref_axis',(0.,0.,-1.));
#12551=DIRECTION('center_axis',(1.,0.,0.));
#12552=DIRECTION('ref_axis',(0.,0.,-1.));
#12553=DIRECTION('center_axis',(1.,0.,0.));
#12554=DIRECTION('ref_axis',(0.,0.,-1.));
#12555=DIRECTION('',(1.,0.,0.));
#12556=DIRECTION('center_axis',(-1.,0.,0.));
#12557=DIRECTION('ref_axis',(0.,0.,-1.));
#12558=DIRECTION('center_axis',(1.,0.,0.));
#12559=DIRECTION('ref_axis',(0.,0.,-1.));
#12560=DIRECTION('center_axis',(1.,0.,0.));
#12561=DIRECTION('ref_axis',(0.,0.,-1.));
#12562=DIRECTION('',(1.,0.,0.));
#12563=DIRECTION('center_axis',(-1.,0.,0.));
#12564=DIRECTION('ref_axis',(0.,0.,-1.));
#12565=DIRECTION('center_axis',(1.,0.,0.));
#12566=DIRECTION('ref_axis',(0.,0.,-1.));
#12567=DIRECTION('center_axis',(1.,0.,0.));
#12568=DIRECTION('ref_axis',(0.,0.,-1.));
#12569=DIRECTION('',(1.,0.,0.));
#12570=DIRECTION('center_axis',(-1.,0.,0.));
#12571=DIRECTION('ref_axis',(0.,0.,-1.));
#12572=DIRECTION('center_axis',(0.,1.,0.));
#12573=DIRECTION('ref_axis',(-1.,0.,0.));
#12574=DIRECTION('',(-1.,0.,0.));
#12575=DIRECTION('',(0.,0.,1.));
#12576=DIRECTION('',(-1.,0.,0.));
#12577=DIRECTION('',(0.,0.,1.));
#12578=DIRECTION('center_axis',(1.,0.,0.));
#12579=DIRECTION('ref_axis',(0.,1.,0.));
#12580=DIRECTION('',(0.,1.,0.));
#12581=DIRECTION('',(0.,1.,0.));
#12582=DIRECTION('',(0.,0.,1.));
#12583=DIRECTION('center_axis',(0.,-1.,0.));
#12584=DIRECTION('ref_axis',(1.,0.,0.));
#12585=DIRECTION('',(1.,0.,0.));
#12586=DIRECTION('',(1.,0.,0.));
#12587=DIRECTION('',(0.,0.,1.));
#12588=DIRECTION('center_axis',(-1.,0.,0.));
#12589=DIRECTION('ref_axis',(0.,-1.,0.));
#12590=DIRECTION('',(0.,-1.,0.));
#12591=DIRECTION('',(0.,-1.,0.));
#12592=DIRECTION('center_axis',(0.,0.,1.));
#12593=DIRECTION('ref_axis',(1.,0.,0.));
#12594=DIRECTION('center_axis',(0.,0.,1.));
#12595=DIRECTION('ref_axis',(1.,0.,0.));
#15593=CARTESIAN_POINT('',(0.,0.,0.));
#15594=CARTESIAN_POINT('Origin',(5.4,2.5,7.8));
#15595=CARTESIAN_POINT('',(5.5,2.5,7.965));
#15596=CARTESIAN_POINT('Origin',(5.5,2.5,7.8));
#15597=CARTESIAN_POINT('',(6.9,2.5,7.965));
#15598=CARTESIAN_POINT('',(5.4,2.5,7.965));
#15599=CARTESIAN_POINT('Origin',(6.9,2.5,7.8));
#15600=CARTESIAN_POINT('Origin',(6.9,2.5,7.8));
#15601=CARTESIAN_POINT('Origin',(5.4,-2.5,9.2));
#15602=CARTESIAN_POINT('',(5.5,-2.5,9.365));
#15603=CARTESIAN_POINT('Origin',(5.5,-2.5,9.2));
#15604=CARTESIAN_POINT('',(6.9,-2.5,9.365));
#15605=CARTESIAN_POINT('',(5.4,-2.5,9.365));
#15606=CARTESIAN_POINT('Origin',(6.9,-2.5,9.2));
#15607=CARTESIAN_POINT('Origin',(6.9,-2.5,9.2));
#15608=CARTESIAN_POINT('Origin',(5.4,-2.5,7.8));
#15609=CARTESIAN_POINT('',(5.5,-2.5,7.965));
#15610=CARTESIAN_POINT('Origin',(5.5,-2.5,7.8));
#15611=CARTESIAN_POINT('',(6.9,-2.5,7.965));
#15612=CARTESIAN_POINT('',(5.4,-2.5,7.965));
#15613=CARTESIAN_POINT('Origin',(6.9,-2.5,7.8));
#15614=CARTESIAN_POINT('Origin',(6.9,-2.5,7.8));
#15615=CARTESIAN_POINT('Origin',(5.4,2.5,9.2));
#15616=CARTESIAN_POINT('',(5.5,2.5,9.365));
#15617=CARTESIAN_POINT('Origin',(5.5,2.5,9.2));
#15618=CARTESIAN_POINT('',(6.9,2.5,9.365));
#15619=CARTESIAN_POINT('',(5.4,2.5,9.365));
#15620=CARTESIAN_POINT('Origin',(6.9,2.5,9.2));
#15621=CARTESIAN_POINT('Origin',(6.9,2.5,9.2));
#15622=CARTESIAN_POINT('Origin',(5.4,0.,2.7));
#15623=CARTESIAN_POINT('',(5.5,-2.02066721859313E-17,2.865));
#15624=CARTESIAN_POINT('Origin',(5.5,0.,2.7));
#15625=CARTESIAN_POINT('',(6.4,-2.02066721859313E-17,2.865));
#15626=CARTESIAN_POINT('',(5.4,-2.02066721859313E-17,2.865));
#15627=CARTESIAN_POINT('Origin',(6.4,0.,2.7));
#15628=CARTESIAN_POINT('Origin',(6.4,0.,2.7));
#15629=CARTESIAN_POINT('Origin',(5.4,0.,5.3));
#15630=CARTESIAN_POINT('',(5.5,-2.02066721859313E-17,5.465));
#15631=CARTESIAN_POINT('Origin',(5.5,0.,5.3));
#15632=CARTESIAN_POINT('',(6.4,-2.02066721859313E-17,5.465));
#15633=CARTESIAN_POINT('',(5.4,-2.02066721859313E-17,5.465));
#15634=CARTESIAN_POINT('Origin',(6.4,0.,5.3));
#15635=CARTESIAN_POINT('Origin',(6.4,0.,5.3));
#15636=CARTESIAN_POINT('Origin',(5.4,4.2,3.));
#15637=CARTESIAN_POINT('',(5.5,4.2,3.165));
#15638=CARTESIAN_POINT('Origin',(5.5,4.2,3.));
#15639=CARTESIAN_POINT('',(8.5,4.2,3.165));
#15640=CARTESIAN_POINT('',(5.4,4.2,3.165));
#15641=CARTESIAN_POINT('Origin',(8.5,4.2,3.));
#15642=CARTESIAN_POINT('Origin',(5.4,-4.2,5.8));
#15643=CARTESIAN_POINT('',(5.5,-4.2,5.965));
#15644=CARTESIAN_POINT('Origin',(5.5,-4.2,5.8));
#15645=CARTESIAN_POINT('',(8.5,-4.2,5.965));
#15646=CARTESIAN_POINT('',(5.4,-4.2,5.965));
#15647=CARTESIAN_POINT('Origin',(8.5,-4.2,5.8));
#15648=CARTESIAN_POINT('Origin',(5.4,-4.2,3.));
#15649=CARTESIAN_POINT('',(5.5,-4.2,3.165));
#15650=CARTESIAN_POINT('Origin',(5.5,-4.2,3.));
#15651=CARTESIAN_POINT('',(8.5,-4.2,3.165));
#15652=CARTESIAN_POINT('',(5.4,-4.2,3.165));
#15653=CARTESIAN_POINT('Origin',(8.5,-4.2,3.));
#15654=CARTESIAN_POINT('Origin',(5.4,4.2,5.8));
#15655=CARTESIAN_POINT('',(5.5,4.2,5.965));
#15656=CARTESIAN_POINT('Origin',(5.5,4.2,5.8));
#15657=CARTESIAN_POINT('',(8.5,4.2,5.965));
#15658=CARTESIAN_POINT('',(5.4,4.2,5.965));
#15659=CARTESIAN_POINT('Origin',(8.5,4.2,5.8));
#15660=CARTESIAN_POINT('Origin',(5.4,0.,4.));
#15661=CARTESIAN_POINT('',(5.5,-1.34711147906209E-16,5.1));
#15662=CARTESIAN_POINT('Origin',(5.5,0.,4.));
#15663=CARTESIAN_POINT('',(8.5,1.34711147906209E-16,5.1));
#15664=CARTESIAN_POINT('',(5.4,-1.34711147906209E-16,5.1));
#15665=CARTESIAN_POINT('Origin',(8.5,0.,4.));
#15666=CARTESIAN_POINT('Origin',(5.4,-3.,4.));
#15667=CARTESIAN_POINT('',(5.5,-3.,5.05));
#15668=CARTESIAN_POINT('Origin',(5.5,-3.,4.));
#15669=CARTESIAN_POINT('',(8.5,-3.,5.05));
#15670=CARTESIAN_POINT('',(5.4,-3.,5.05));
#15671=CARTESIAN_POINT('Origin',(8.5,-3.,4.));
#15672=CARTESIAN_POINT('Origin',(5.4,3.,4.));
#15673=CARTESIAN_POINT('',(5.5,3.,5.05));
#15674=CARTESIAN_POINT('Origin',(5.5,3.,4.));
#15675=CARTESIAN_POINT('',(8.5,3.,5.05));
#15676=CARTESIAN_POINT('',(5.4,3.,5.05));
#15677=CARTESIAN_POINT('Origin',(8.5,3.,4.));
#15678=CARTESIAN_POINT('Origin',(8.5,4.7,2.3));
#15679=CARTESIAN_POINT('',(8.5,4.7,2.3));
#15680=CARTESIAN_POINT('',(5.5,4.7,2.3));
#15681=CARTESIAN_POINT('',(8.5,4.7,2.3));
#15682=CARTESIAN_POINT('',(5.5,4.7,10.));
#15683=CARTESIAN_POINT('',(5.5,4.7,2.3));
#15684=CARTESIAN_POINT('',(8.5,4.7,10.));
#15685=CARTESIAN_POINT('',(8.5,4.7,10.));
#15686=CARTESIAN_POINT('',(8.5,4.7,2.3));
#15687=CARTESIAN_POINT('Origin',(8.5,-4.7,2.3));
#15688=CARTESIAN_POINT('',(8.5,-4.7,2.3));
#15689=CARTESIAN_POINT('',(8.5,-4.7,2.3));
#15690=CARTESIAN_POINT('',(8.5,-4.7,10.));
#15691=CARTESIAN_POINT('',(8.5,-4.7,10.));
#15692=CARTESIAN_POINT('',(8.5,-4.7,2.3));
#15693=CARTESIAN_POINT('Origin',(5.5,-4.7,2.3));
#15694=CARTESIAN_POINT('',(5.5,-4.7,2.3));
#15695=CARTESIAN_POINT('',(5.5,-4.7,2.3));
#15696=CARTESIAN_POINT('',(5.5,-4.7,10.));
#15697=CARTESIAN_POINT('',(5.5,-4.7,10.));
#15698=CARTESIAN_POINT('',(5.5,-4.7,2.3));
#15699=CARTESIAN_POINT('Origin',(5.5,4.7,2.3));
#15700=CARTESIAN_POINT('',(5.5,4.7,2.3));
#15701=CARTESIAN_POINT('',(5.5,4.7,10.));
#15702=CARTESIAN_POINT('Origin',(7.,0.,10.));
#15703=CARTESIAN_POINT('Origin',(7.,0.,2.3));
#16731=UNCERTAINTY_MEASURE_WITH_UNIT(LENGTH_MEASURE(0.001),#16800,
'DISTANCE_ACCURACY_VALUE',
'Maximum model space distance between geometric entities at asserted c
onnectivities');
#16750=UNCERTAINTY_MEASURE_WITH_UNIT(LENGTH_MEASURE(0.001),#16800,
'DISTANCE_ACCURACY_VALUE',
'Maximum model space distance between geometric entities at asserted c
onnectivities');
#16780=(
GEOMETRIC_REPRESENTATION_CONTEXT(3)
GLOBAL_UNCERTAINTY_ASSIGNED_CONTEXT((#16731))
GLOBAL_UNIT_ASSIGNED_CONTEXT((#16800,#16802,#16803))
REPRESENTATION_CONTEXT('','3D')
);
#16799=(
GEOMETRIC_REPRESENTATION_CONTEXT(3)
GLOBAL_UNCERTAINTY_ASSIGNED_CONTEXT((#16750))
GLOBAL_UNIT_ASSIGNED_CONTEXT((#16800,#16802,#16803))
REPRESENTATION_CONTEXT('','3D')
);
#16800=(
LENGTH_UNIT()
NAMED_UNIT(*)
SI_UNIT(.CENTI.,.METRE.)
);
#16802=(
NAMED_UNIT(*)
PLANE_ANGLE_UNIT()
SI_UNIT($,.RADIAN.)
);
#16803=(
NAMED_UNIT(*)
SI_UNIT($,.STERADIAN.)
SOLID_ANGLE_UNIT()
);
#16833=SHAPE_DEFINITION_REPRESENTATION(#16886,#17042);
#16886=PRODUCT_DEFINITION_SHAPE('',$,#17091);
#17042=SHAPE_REPRESENTATION('',(#10256),#16780);
#17061=PRODUCT_DEFINITION_CONTEXT('part definition',#17207,'design');
#17091=PRODUCT_DEFINITION('Right jaw body','Right jaw body',#17139,#17061);
#17139=PRODUCT_DEFINITION_FORMATION('',$,#17238);
#17207=APPLICATION_CONTEXT(
'Core Data for Automotive Mechanical Design Process');
#17208=PRODUCT_CONTEXT('part definition',#17207,'mechanical');
#17238=PRODUCT('Right jaw body','Right jaw body','Right jaw body',(#17208));
#17299=COLOUR_RGB('Dark Blue',0.08,0.2,0.34);
#17300=FILL_AREA_STYLE_COLOUR('',#17299);
#17301=FILL_AREA_STYLE('',(#17300));
#17302=SURFACE_STYLE_FILL_AREA(#17301);
#17303=SURFACE_SIDE_STYLE('',(#17302));
#17304=SURFACE_STYLE_USAGE(.BOTH.,#17303);
#17305=PRESENTATION_STYLE_ASSIGNMENT((#17304));
ENDSEC;
END-ISO-10303-21;
